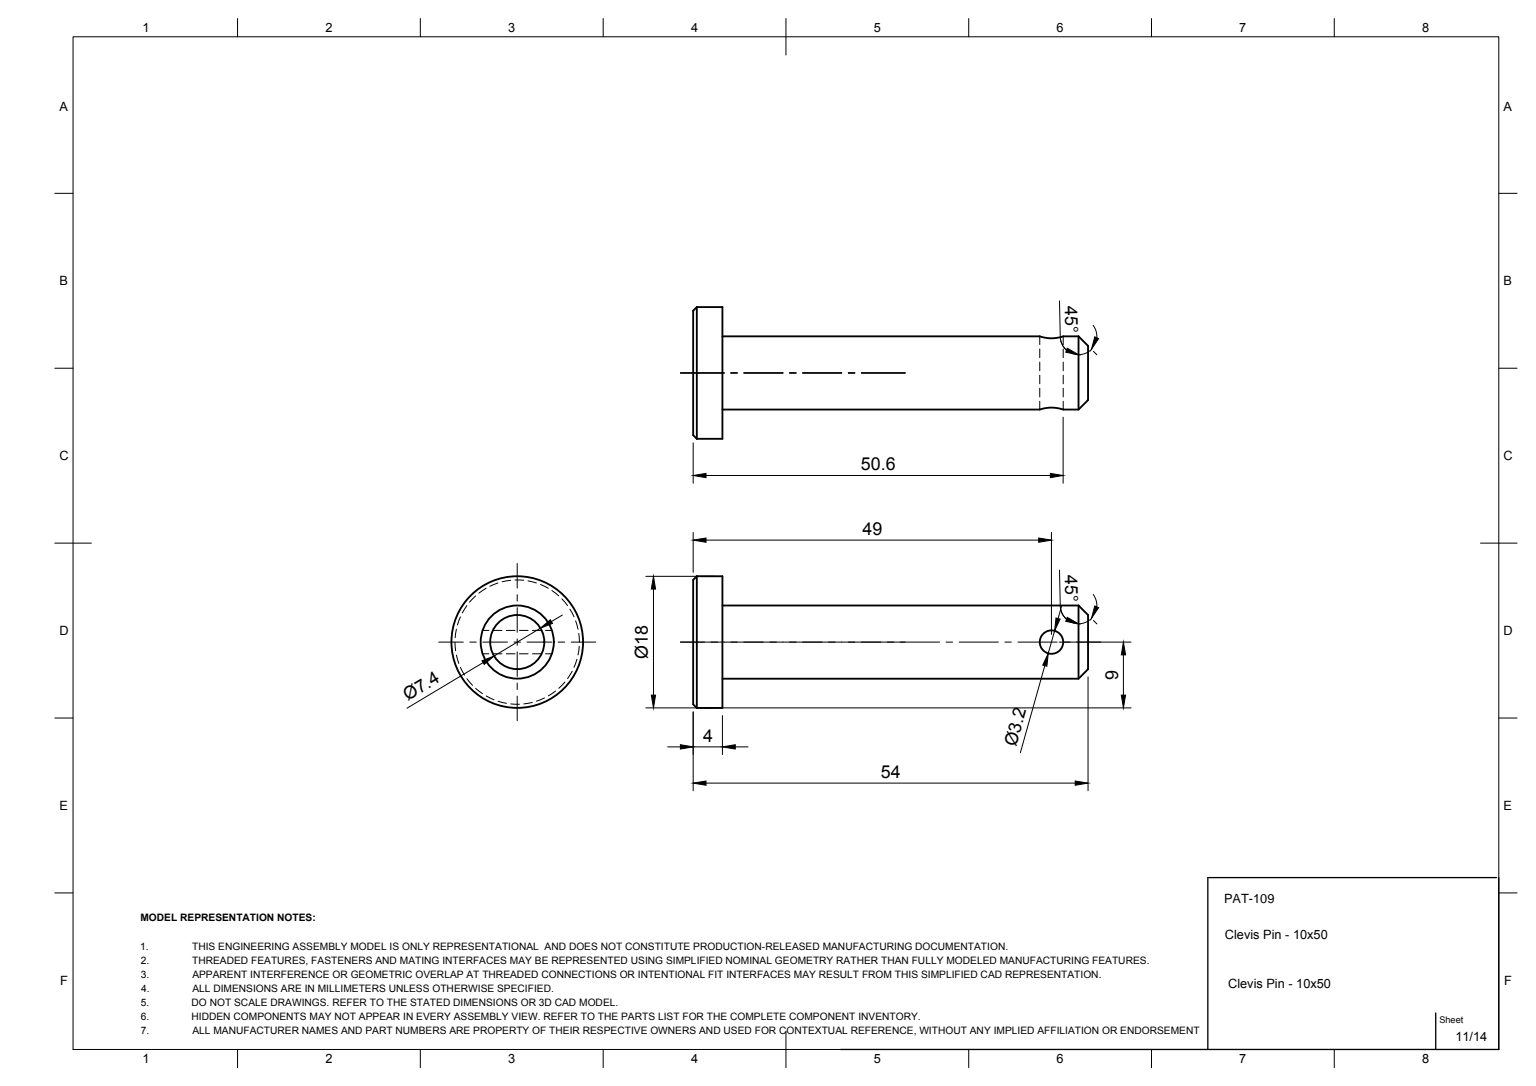
ISO-10303-21;
HEADER;
/* Generated by software containing ST-Developer
 * from STEP Tools, Inc. (www.steptools.com) 
 */

FILE_DESCRIPTION(
/* description */ ('Twin-shackle spreader bar'),
/* implementation_level */ '2;1');

FILE_NAME(
/* name */ 'Clevis Pin - 10x50.step',
/* time_stamp */ '2026-10-27T20:18:10-07:00',
/* author */ (''),
/* organization */ (''),
/* preprocessor_version */ 'ST-DEVELOPER v20.2',
/* originating_system */ 'Autodesk Translation Framework v15.17.0.0',
/* authorisation */ '');

FILE_SCHEMA (('AUTOMOTIVE_DESIGN { 1 0 10303 214 3 1 1 }'));
ENDSEC;

DATA;
#10=MECHANICAL_DESIGN_GEOMETRIC_PRESENTATION_REPRESENTATION('',(#161),#1829);
#12=CONICAL_SURFACE('',#1083,0.875,0.785398163397448);
#13=CONICAL_SURFACE('',#1091,0.435,0.785398163397449);
#14=B_SPLINE_CURVE_WITH_KNOTS('',3,(#1599,#1600,#1601,#1602,#1603,#1604,
#1605,#1606,#1607,#1608),.UNSPECIFIED.,.F.,.F.,(4,2,2,2,4),(0.,0.0607460470679908,
0.121492094135982,0.182214421454286,0.242936748772591),.UNSPECIFIED.);
#15=B_SPLINE_CURVE_WITH_KNOTS('',3,(#1611,#1612,#1613,#1614,#1615,#1616,
#1617,#1618,#1619,#1620,#1621,#1622,#1623,#1624,#1625,#1626,#1627,#1628,
#1629,#1630,#1631,#1632,#1633,#1634,#1635,#1636,#1637,#1638,#1639,#1640,
#1641,#1642,#1643,#1644),.UNSPECIFIED.,.T.,.F.,(4,2,2,2,2,2,2,2,2,2,2,2,
2,2,2,2,4),(0.,0.0607460470679913,0.121492094135983,0.182214421454287,0.242936748772591,
0.303659076090896,0.3643814034092,0.425127450477191,0.485873497545182,0.546619544613173,
0.607365591681164,0.668087918999469,0.728810246317773,0.789532573636077,
0.850254900954382,0.911000948022373,0.971746995090363),.UNSPECIFIED.);
#16=B_SPLINE_CURVE_WITH_KNOTS('',3,(#1646,#1647,#1648,#1649,#1650,#1651,
#1652,#1653,#1654,#1655),.UNSPECIFIED.,.F.,.F.,(4,2,2,2,4),(0.728810246317772,
0.789532573636077,0.850254900954381,0.911000948022372,0.971746995090363),
 .UNSPECIFIED.);
#17=B_SPLINE_CURVE_WITH_KNOTS('',3,(#1656,#1657,#1658,#1659,#1660,#1661,
#1662,#1663,#1664,#1665,#1666,#1667,#1668,#1669,#1670,#1671,#1672,#1673),
 .UNSPECIFIED.,.F.,.F.,(4,2,2,2,2,2,2,2,4),(0.242936748772591,0.303659076090895,
0.364381403409199,0.42512745047719,0.485873497545182,0.546619544613173,
0.607365591681163,0.668087918999468,0.728810246317772),.UNSPECIFIED.);
#116=CIRCLE('',#1082,0.85);
#117=CIRCLE('',#1084,0.9);
#118=CIRCLE('',#1086,0.9);
#119=CIRCLE('',#1088,0.5);
#120=CIRCLE('',#1090,0.5);
#121=CIRCLE('',#1092,0.37);
#137=CYLINDRICAL_SURFACE('',#1080,0.16);
#138=CYLINDRICAL_SURFACE('',#1085,0.9);
#139=CYLINDRICAL_SURFACE('',#1089,0.5);
#147=SHAPE_REPRESENTATION_RELATIONSHIP('SRR','None',#1885,#154);
#154=ADVANCED_BREP_SHAPE_REPRESENTATION('',(#168),#1826);
#161=STYLED_ITEM('',(#1984),#168);
#168=MANIFOLD_SOLID_BREP('Body1',#941);
#181=FACE_BOUND('',#284,.T.);
#182=FACE_BOUND('',#286,.T.);
#219=FACE_OUTER_BOUND('',#279,.T.);
#220=FACE_OUTER_BOUND('',#280,.T.);
#221=FACE_OUTER_BOUND('',#281,.T.);
#222=FACE_OUTER_BOUND('',#282,.T.);
#223=FACE_OUTER_BOUND('',#283,.T.);
#224=FACE_OUTER_BOUND('',#285,.T.);
#225=FACE_OUTER_BOUND('',#287,.T.);
#226=FACE_OUTER_BOUND('',#288,.T.);
#279=EDGE_LOOP('',(#784,#785,#786,#787,#788,#789));
#280=EDGE_LOOP('',(#790));
#281=EDGE_LOOP('',(#791,#792,#793,#794));
#282=EDGE_LOOP('',(#795,#796,#797,#798));
#283=EDGE_LOOP('',(#799));
#284=EDGE_LOOP('',(#800));
#285=EDGE_LOOP('',(#801,#802,#803,#804,#805,#806,#807,#808,#809));
#286=EDGE_LOOP('',(#810));
#287=EDGE_LOOP('',(#811,#812,#813,#814));
#288=EDGE_LOOP('',(#815));
#364=LINE('',#1610,#440);
#365=LINE('',#1680,#441);
#366=LINE('',#1684,#442);
#367=LINE('',#1691,#443);
#368=LINE('',#1692,#444);
#369=LINE('',#1696,#445);
#440=VECTOR('',#1312,0.16);
#441=VECTOR('',#1321,0.875);
#442=VECTOR('',#1326,0.9);
#443=VECTOR('',#1335,0.5);
#444=VECTOR('',#1336,0.5);
#445=VECTOR('',#1341,0.435);
#503=VERTEX_POINT('',#1597);
#504=VERTEX_POINT('',#1598);
#505=VERTEX_POINT('',#1609);
#506=VERTEX_POINT('',#1645);
#507=VERTEX_POINT('',#1675);
#508=VERTEX_POINT('',#1678);
#509=VERTEX_POINT('',#1682);
#510=VERTEX_POINT('',#1686);
#511=VERTEX_POINT('',#1689);
#512=VERTEX_POINT('',#1694);
#600=EDGE_CURVE('',#503,#504,#14,.T.);
#601=EDGE_CURVE('',#503,#505,#364,.T.);
#602=EDGE_CURVE('',#505,#505,#15,.T.);
#603=EDGE_CURVE('',#506,#503,#16,.T.);
#604=EDGE_CURVE('',#504,#506,#17,.T.);
#605=EDGE_CURVE('',#507,#507,#116,.T.);
#606=EDGE_CURVE('',#508,#508,#117,.T.);
#607=EDGE_CURVE('',#508,#507,#365,.T.);
#608=EDGE_CURVE('',#509,#509,#118,.T.);
#609=EDGE_CURVE('',#509,#508,#366,.T.);
#610=EDGE_CURVE('',#510,#510,#119,.T.);
#611=EDGE_CURVE('',#511,#511,#120,.T.);
#612=EDGE_CURVE('',#511,#504,#367,.T.);
#613=EDGE_CURVE('',#506,#510,#368,.T.);
#614=EDGE_CURVE('',#512,#512,#121,.T.);
#615=EDGE_CURVE('',#512,#511,#369,.T.);
#784=ORIENTED_EDGE('',*,*,#600,.F.);
#785=ORIENTED_EDGE('',*,*,#601,.T.);
#786=ORIENTED_EDGE('',*,*,#602,.F.);
#787=ORIENTED_EDGE('',*,*,#601,.F.);
#788=ORIENTED_EDGE('',*,*,#603,.F.);
#789=ORIENTED_EDGE('',*,*,#604,.F.);
#790=ORIENTED_EDGE('',*,*,#605,.F.);
#791=ORIENTED_EDGE('',*,*,#606,.F.);
#792=ORIENTED_EDGE('',*,*,#607,.T.);
#793=ORIENTED_EDGE('',*,*,#605,.T.);
#794=ORIENTED_EDGE('',*,*,#607,.F.);
#795=ORIENTED_EDGE('',*,*,#608,.F.);
#796=ORIENTED_EDGE('',*,*,#609,.T.);
#797=ORIENTED_EDGE('',*,*,#606,.T.);
#798=ORIENTED_EDGE('',*,*,#609,.F.);
#799=ORIENTED_EDGE('',*,*,#608,.T.);
#800=ORIENTED_EDGE('',*,*,#610,.F.);
#801=ORIENTED_EDGE('',*,*,#611,.F.);
#802=ORIENTED_EDGE('',*,*,#612,.T.);
#803=ORIENTED_EDGE('',*,*,#604,.T.);
#804=ORIENTED_EDGE('',*,*,#613,.T.);
#805=ORIENTED_EDGE('',*,*,#610,.T.);
#806=ORIENTED_EDGE('',*,*,#613,.F.);
#807=ORIENTED_EDGE('',*,*,#603,.T.);
#808=ORIENTED_EDGE('',*,*,#600,.T.);
#809=ORIENTED_EDGE('',*,*,#612,.F.);
#810=ORIENTED_EDGE('',*,*,#602,.T.);
#811=ORIENTED_EDGE('',*,*,#614,.F.);
#812=ORIENTED_EDGE('',*,*,#615,.T.);
#813=ORIENTED_EDGE('',*,*,#611,.T.);
#814=ORIENTED_EDGE('',*,*,#615,.F.);
#815=ORIENTED_EDGE('',*,*,#614,.T.);
#879=PLANE('',#1081);
#880=PLANE('',#1087);
#881=PLANE('',#1093);
#920=ADVANCED_FACE('',(#219),#137,.F.);
#921=ADVANCED_FACE('',(#220),#879,.T.);
#922=ADVANCED_FACE('',(#221),#12,.T.);
#923=ADVANCED_FACE('',(#222),#138,.T.);
#924=ADVANCED_FACE('',(#223,#181),#880,.T.);
#925=ADVANCED_FACE('',(#224,#182),#139,.T.);
#926=ADVANCED_FACE('',(#225),#13,.T.);
#927=ADVANCED_FACE('',(#226),#881,.T.);
#941=CLOSED_SHELL('',(#920,#921,#922,#923,#924,#925,#926,#927));
#1079=AXIS2_PLACEMENT_3D('',#1595,#1308,#1309);
#1080=AXIS2_PLACEMENT_3D('',#1596,#1310,#1311);
#1081=AXIS2_PLACEMENT_3D('',#1674,#1313,#1314);
#1082=AXIS2_PLACEMENT_3D('',#1676,#1315,#1316);
#1083=AXIS2_PLACEMENT_3D('',#1677,#1317,#1318);
#1084=AXIS2_PLACEMENT_3D('',#1679,#1319,#1320);
#1085=AXIS2_PLACEMENT_3D('',#1681,#1322,#1323);
#1086=AXIS2_PLACEMENT_3D('',#1683,#1324,#1325);
#1087=AXIS2_PLACEMENT_3D('',#1685,#1327,#1328);
#1088=AXIS2_PLACEMENT_3D('',#1687,#1329,#1330);
#1089=AXIS2_PLACEMENT_3D('',#1688,#1331,#1332);
#1090=AXIS2_PLACEMENT_3D('',#1690,#1333,#1334);
#1091=AXIS2_PLACEMENT_3D('',#1693,#1337,#1338);
#1092=AXIS2_PLACEMENT_3D('',#1695,#1339,#1340);
#1093=AXIS2_PLACEMENT_3D('',#1697,#1342,#1343);
#1308=DIRECTION('axis',(0.,0.,1.));
#1309=DIRECTION('refdir',(1.,0.,0.));
#1310=DIRECTION('center_axis',(1.,0.,0.));
#1311=DIRECTION('ref_axis',(0.,0.,-1.));
#1312=DIRECTION('',(1.,0.,0.));
#1313=DIRECTION('center_axis',(0.,1.,0.));
#1314=DIRECTION('ref_axis',(0.,0.,1.));
#1315=DIRECTION('center_axis',(0.,-1.,0.));
#1316=DIRECTION('ref_axis',(1.,0.,0.));
#1317=DIRECTION('center_axis',(0.,-1.,0.));
#1318=DIRECTION('ref_axis',(1.,0.,0.));
#1319=DIRECTION('center_axis',(0.,-1.,0.));
#1320=DIRECTION('ref_axis',(1.,0.,0.));
#1321=DIRECTION('',(0.707106781186548,0.707106781186547,8.65956056235494E-17));
#1322=DIRECTION('center_axis',(0.,-1.,0.));
#1323=DIRECTION('ref_axis',(1.,0.,0.));
#1324=DIRECTION('center_axis',(0.,-1.,0.));
#1325=DIRECTION('ref_axis',(1.,0.,0.));
#1326=DIRECTION('',(0.,1.,0.));
#1327=DIRECTION('center_axis',(0.,-1.,0.));
#1328=DIRECTION('ref_axis',(0.,0.,-1.));
#1329=DIRECTION('center_axis',(0.,-1.,0.));
#1330=DIRECTION('ref_axis',(1.,0.,0.));
#1331=DIRECTION('center_axis',(0.,-1.,0.));
#1332=DIRECTION('ref_axis',(1.,0.,0.));
#1333=DIRECTION('center_axis',(0.,-1.,0.));
#1334=DIRECTION('ref_axis',(1.,0.,0.));
#1335=DIRECTION('',(0.,1.,0.));
#1336=DIRECTION('',(0.,1.,0.));
#1337=DIRECTION('center_axis',(0.,1.,0.));
#1338=DIRECTION('ref_axis',(1.,0.,0.));
#1339=DIRECTION('center_axis',(0.,-1.,0.));
#1340=DIRECTION('ref_axis',(1.,0.,0.));
#1341=DIRECTION('',(-0.707106781186548,0.707106781186547,-8.65956056235493E-17));
#1342=DIRECTION('center_axis',(0.,-1.,0.));
#1343=DIRECTION('ref_axis',(0.,0.,-1.));
#1595=CARTESIAN_POINT('',(0.,0.,0.));
#1596=CARTESIAN_POINT('Origin',(0.,-4.5,0.));
#1597=CARTESIAN_POINT('',(-0.47370877129308,-4.5,0.16));
#1598=CARTESIAN_POINT('',(-0.5,-4.66,-2.19425525987998E-17));
#1599=CARTESIAN_POINT('Ctrl Pts',(-0.47370877129308,-4.5,0.16));
#1600=CARTESIAN_POINT('Ctrl Pts',(-0.47370877129308,-4.520248682356,0.16));
#1601=CARTESIAN_POINT('Ctrl Pts',(-0.47514325949633,-4.54174042142149,0.155923994634429));
#1602=CARTESIAN_POINT('Ctrl Pts',(-0.480206450087542,-4.58111342508711,
0.13955347049286));
#1603=CARTESIAN_POINT('Ctrl Pts',(-0.483749754411139,-4.59900844138689,
0.127265728592806));
#1604=CARTESIAN_POINT('Ctrl Pts',(-0.490312616976052,-4.62726021172536,
0.0990139582543377));
#1605=CARTESIAN_POINT('Ctrl Pts',(-0.493774986141774,-4.6395522112502,0.0811167261268817));
#1606=CARTESIAN_POINT('Ctrl Pts',(-0.498649979553188,-4.65592589713458,
0.0417355732628882));
#1607=CARTESIAN_POINT('Ctrl Pts',(-0.5,-4.66,0.0202407757727682));
#1608=CARTESIAN_POINT('Ctrl Pts',(-0.5,-4.66,-2.42861286636753E-17));
#1609=CARTESIAN_POINT('',(0.47370877129308,-4.5,0.16));
#1610=CARTESIAN_POINT('',(0.,-4.5,0.16));
#1611=CARTESIAN_POINT('Ctrl Pts',(0.47370877129308,-4.5,0.16));
#1612=CARTESIAN_POINT('Ctrl Pts',(0.47370877129308,-4.479751317644,0.16));
#1613=CARTESIAN_POINT('Ctrl Pts',(0.47514325949633,-4.45825957857851,0.155923994634429));
#1614=CARTESIAN_POINT('Ctrl Pts',(0.480206450087542,-4.41888657491289,0.139553470492859));
#1615=CARTESIAN_POINT('Ctrl Pts',(0.483749754411139,-4.40099155861311,0.127265728592806));
#1616=CARTESIAN_POINT('Ctrl Pts',(0.490312616976052,-4.37273978827464,0.0990139582543375));
#1617=CARTESIAN_POINT('Ctrl Pts',(0.493774986141774,-4.3604477887498,0.0811167261268814));
#1618=CARTESIAN_POINT('Ctrl Pts',(0.498649979553188,-4.34407410286542,0.0417355732628877));
#1619=CARTESIAN_POINT('Ctrl Pts',(0.5,-4.34,0.020240775772768));
#1620=CARTESIAN_POINT('Ctrl Pts',(0.5,-4.34,-0.0202407757727682));
#1621=CARTESIAN_POINT('Ctrl Pts',(0.498649979553188,-4.34407410286542,-0.0417355732628882));
#1622=CARTESIAN_POINT('Ctrl Pts',(0.493774986141774,-4.3604477887498,-0.0811167261268817));
#1623=CARTESIAN_POINT('Ctrl Pts',(0.490312616976052,-4.37273978827464,-0.0990139582543377));
#1624=CARTESIAN_POINT('Ctrl Pts',(0.483749754411139,-4.40099155861311,-0.127265728592806));
#1625=CARTESIAN_POINT('Ctrl Pts',(0.480206450087542,-4.41888657491289,-0.13955347049286));
#1626=CARTESIAN_POINT('Ctrl Pts',(0.47514325949633,-4.45825957857851,-0.155923994634429));
#1627=CARTESIAN_POINT('Ctrl Pts',(0.47370877129308,-4.479751317644,-0.16));
#1628=CARTESIAN_POINT('Ctrl Pts',(0.47370877129308,-4.520248682356,-0.16));
#1629=CARTESIAN_POINT('Ctrl Pts',(0.47514325949633,-4.54174042142149,-0.155923994634429));
#1630=CARTESIAN_POINT('Ctrl Pts',(0.480206450087542,-4.58111342508711,-0.139553470492859));
#1631=CARTESIAN_POINT('Ctrl Pts',(0.483749754411139,-4.59900844138689,-0.127265728592806));
#1632=CARTESIAN_POINT('Ctrl Pts',(0.490312616976052,-4.62726021172536,-0.0990139582543375));
#1633=CARTESIAN_POINT('Ctrl Pts',(0.493774986141774,-4.6395522112502,-0.0811167261268813));
#1634=CARTESIAN_POINT('Ctrl Pts',(0.498649979553188,-4.65592589713458,-0.041735573262888));
#1635=CARTESIAN_POINT('Ctrl Pts',(0.5,-4.66,-0.0202407757727681));
#1636=CARTESIAN_POINT('Ctrl Pts',(0.5,-4.66,0.0202407757727682));
#1637=CARTESIAN_POINT('Ctrl Pts',(0.498649979553188,-4.65592589713458,0.0417355732628882));
#1638=CARTESIAN_POINT('Ctrl Pts',(0.493774986141774,-4.6395522112502,0.0811167261268817));
#1639=CARTESIAN_POINT('Ctrl Pts',(0.490312616976052,-4.62726021172536,0.0990139582543377));
#1640=CARTESIAN_POINT('Ctrl Pts',(0.483749754411139,-4.59900844138689,0.127265728592806));
#1641=CARTESIAN_POINT('Ctrl Pts',(0.480206450087542,-4.58111342508711,0.13955347049286));
#1642=CARTESIAN_POINT('Ctrl Pts',(0.47514325949633,-4.54174042142149,0.155923994634429));
#1643=CARTESIAN_POINT('Ctrl Pts',(0.47370877129308,-4.520248682356,0.16));
#1644=CARTESIAN_POINT('Ctrl Pts',(0.47370877129308,-4.5,0.16));
#1645=CARTESIAN_POINT('',(-0.5,-4.34,-4.01571490965563E-17));
#1646=CARTESIAN_POINT('Ctrl Pts',(-0.5,-4.34,-2.08166817117217E-17));
#1647=CARTESIAN_POINT('Ctrl Pts',(-0.5,-4.34,0.0202407757727681));
#1648=CARTESIAN_POINT('Ctrl Pts',(-0.498649979553188,-4.34407410286542,
0.041735573262888));
#1649=CARTESIAN_POINT('Ctrl Pts',(-0.493774986141774,-4.3604477887498,0.0811167261268813));
#1650=CARTESIAN_POINT('Ctrl Pts',(-0.490312616976052,-4.37273978827464,
0.0990139582543375));
#1651=CARTESIAN_POINT('Ctrl Pts',(-0.483749754411139,-4.40099155861311,
0.127265728592806));
#1652=CARTESIAN_POINT('Ctrl Pts',(-0.480206450087542,-4.41888657491289,
0.139553470492859));
#1653=CARTESIAN_POINT('Ctrl Pts',(-0.47514325949633,-4.45825957857851,0.155923994634429));
#1654=CARTESIAN_POINT('Ctrl Pts',(-0.47370877129308,-4.479751317644,0.16));
#1655=CARTESIAN_POINT('Ctrl Pts',(-0.47370877129308,-4.5,0.16));
#1656=CARTESIAN_POINT('Ctrl Pts',(-0.5,-4.66,1.38777878078145E-17));
#1657=CARTESIAN_POINT('Ctrl Pts',(-0.5,-4.66,-0.0202407757727681));
#1658=CARTESIAN_POINT('Ctrl Pts',(-0.498649979553188,-4.65592589713458,
-0.041735573262888));
#1659=CARTESIAN_POINT('Ctrl Pts',(-0.493774986141774,-4.6395522112502,-0.0811167261268813));
#1660=CARTESIAN_POINT('Ctrl Pts',(-0.490312616976052,-4.62726021172536,
-0.0990139582543375));
#1661=CARTESIAN_POINT('Ctrl Pts',(-0.483749754411139,-4.59900844138689,
-0.127265728592806));
#1662=CARTESIAN_POINT('Ctrl Pts',(-0.480206450087542,-4.58111342508711,
-0.139553470492859));
#1663=CARTESIAN_POINT('Ctrl Pts',(-0.47514325949633,-4.54174042142149,-0.155923994634429));
#1664=CARTESIAN_POINT('Ctrl Pts',(-0.47370877129308,-4.520248682356,-0.16));
#1665=CARTESIAN_POINT('Ctrl Pts',(-0.47370877129308,-4.479751317644,-0.16));
#1666=CARTESIAN_POINT('Ctrl Pts',(-0.47514325949633,-4.45825957857851,-0.155923994634429));
#1667=CARTESIAN_POINT('Ctrl Pts',(-0.480206450087542,-4.41888657491289,
-0.13955347049286));
#1668=CARTESIAN_POINT('Ctrl Pts',(-0.483749754411139,-4.40099155861311,
-0.127265728592806));
#1669=CARTESIAN_POINT('Ctrl Pts',(-0.490312616976052,-4.37273978827464,
-0.0990139582543377));
#1670=CARTESIAN_POINT('Ctrl Pts',(-0.493774986141774,-4.3604477887498,-0.0811167261268817));
#1671=CARTESIAN_POINT('Ctrl Pts',(-0.498649979553188,-4.34407410286542,
-0.0417355732628882));
#1672=CARTESIAN_POINT('Ctrl Pts',(-0.5,-4.34,-0.0202407757727682));
#1673=CARTESIAN_POINT('Ctrl Pts',(-0.5,-4.34,-1.73472347597681E-17));
#1674=CARTESIAN_POINT('Origin',(0.85,0.4,0.));
#1675=CARTESIAN_POINT('',(-0.85,0.4,-1.04094977927525E-16));
#1676=CARTESIAN_POINT('Origin',(0.,0.4,0.));
#1677=CARTESIAN_POINT('Origin',(0.,0.375,0.));
#1678=CARTESIAN_POINT('',(-0.9,0.35,-1.10218211923262E-16));
#1679=CARTESIAN_POINT('Origin',(0.,0.35,0.));
#1680=CARTESIAN_POINT('',(-0.875,0.375,-1.07156594925393E-16));
#1681=CARTESIAN_POINT('Origin',(0.,0.175,0.));
#1682=CARTESIAN_POINT('',(-0.9,0.,-1.10218211923262E-16));
#1683=CARTESIAN_POINT('Origin',(0.,0.,0.));
#1684=CARTESIAN_POINT('',(-0.9,0.175,-1.10218211923262E-16));
#1685=CARTESIAN_POINT('Origin',(0.5,0.,0.));
#1686=CARTESIAN_POINT('',(-0.5,0.,-6.12323399573677E-17));
#1687=CARTESIAN_POINT('Origin',(0.,0.,0.));
#1688=CARTESIAN_POINT('Origin',(0.,-2.435,0.));
#1689=CARTESIAN_POINT('',(-0.5,-4.87,-6.12323399573677E-17));
#1690=CARTESIAN_POINT('Origin',(0.,-4.87,0.));
#1691=CARTESIAN_POINT('',(-0.5,-2.435,-6.12323399573677E-17));
#1692=CARTESIAN_POINT('',(-0.5,-2.435,-6.12323399573677E-17));
#1693=CARTESIAN_POINT('Origin',(0.,-4.935,0.));
#1694=CARTESIAN_POINT('',(-0.37,-5.,-4.53119315684521E-17));
#1695=CARTESIAN_POINT('Origin',(0.,-5.,0.));
#1696=CARTESIAN_POINT('',(-0.435,-4.935,-5.32721357629099E-17));
#1697=CARTESIAN_POINT('Origin',(0.,-5.,0.));
#1814=UNCERTAINTY_MEASURE_WITH_UNIT(LENGTH_MEASURE(0.001),#1830,
'DISTANCE_ACCURACY_VALUE',
'Maximum model space distance between geometric entities at asserted c
onnectivities');
#1817=UNCERTAINTY_MEASURE_WITH_UNIT(LENGTH_MEASURE(0.001),#1830,
'DISTANCE_ACCURACY_VALUE',
'Maximum model space distance between geometric entities at asserted c
onnectivities');
#1826=(
GEOMETRIC_REPRESENTATION_CONTEXT(3)
GLOBAL_UNCERTAINTY_ASSIGNED_CONTEXT((#1814))
GLOBAL_UNIT_ASSIGNED_CONTEXT((#1830,#1832,#1833))
REPRESENTATION_CONTEXT('','3D')
);
#1829=(
GEOMETRIC_REPRESENTATION_CONTEXT(3)
GLOBAL_UNCERTAINTY_ASSIGNED_CONTEXT((#1817))
GLOBAL_UNIT_ASSIGNED_CONTEXT((#1830,#1832,#1833))
REPRESENTATION_CONTEXT('','3D')
);
#1830=(
LENGTH_UNIT()
NAMED_UNIT(*)
SI_UNIT(.CENTI.,.METRE.)
);
#1832=(
NAMED_UNIT(*)
PLANE_ANGLE_UNIT()
SI_UNIT($,.RADIAN.)
);
#1833=(
NAMED_UNIT(*)
SI_UNIT($,.STERADIAN.)
SOLID_ANGLE_UNIT()
);
#1842=SHAPE_DEFINITION_REPRESENTATION(#1857,#1885);
#1857=PRODUCT_DEFINITION_SHAPE('',$,#1897);
#1885=SHAPE_REPRESENTATION('',(#1079),#1826);
#1888=PRODUCT_DEFINITION_CONTEXT('part definition',#1923,'design');
#1897=PRODUCT_DEFINITION('Clevis Pin - 10x50','Clevis Pin - 10x50',#1908,
#1888);
#1908=PRODUCT_DEFINITION_FORMATION('',$,#1933);
#1923=APPLICATION_CONTEXT(
'Core Data for Automotive Mechanical Design Process');
#1924=PRODUCT_CONTEXT('part definition',#1923,'mechanical');
#1933=PRODUCT('Clevis Pin - 10x50','Clevis Pin - 10x50',
'Clevis Pin - 10x50',(#1924));
#1978=COLOUR_RGB('Grey',0.48,0.52,0.57);
#1979=FILL_AREA_STYLE_COLOUR('',#1978);
#1980=FILL_AREA_STYLE('',(#1979));
#1981=SURFACE_STYLE_FILL_AREA(#1980);
#1982=SURFACE_SIDE_STYLE('',(#1981));
#1983=SURFACE_STYLE_USAGE(.BOTH.,#1982);
#1984=PRESENTATION_STYLE_ASSIGNMENT((#1983));
ENDSEC;
END-ISO-10303-21;
